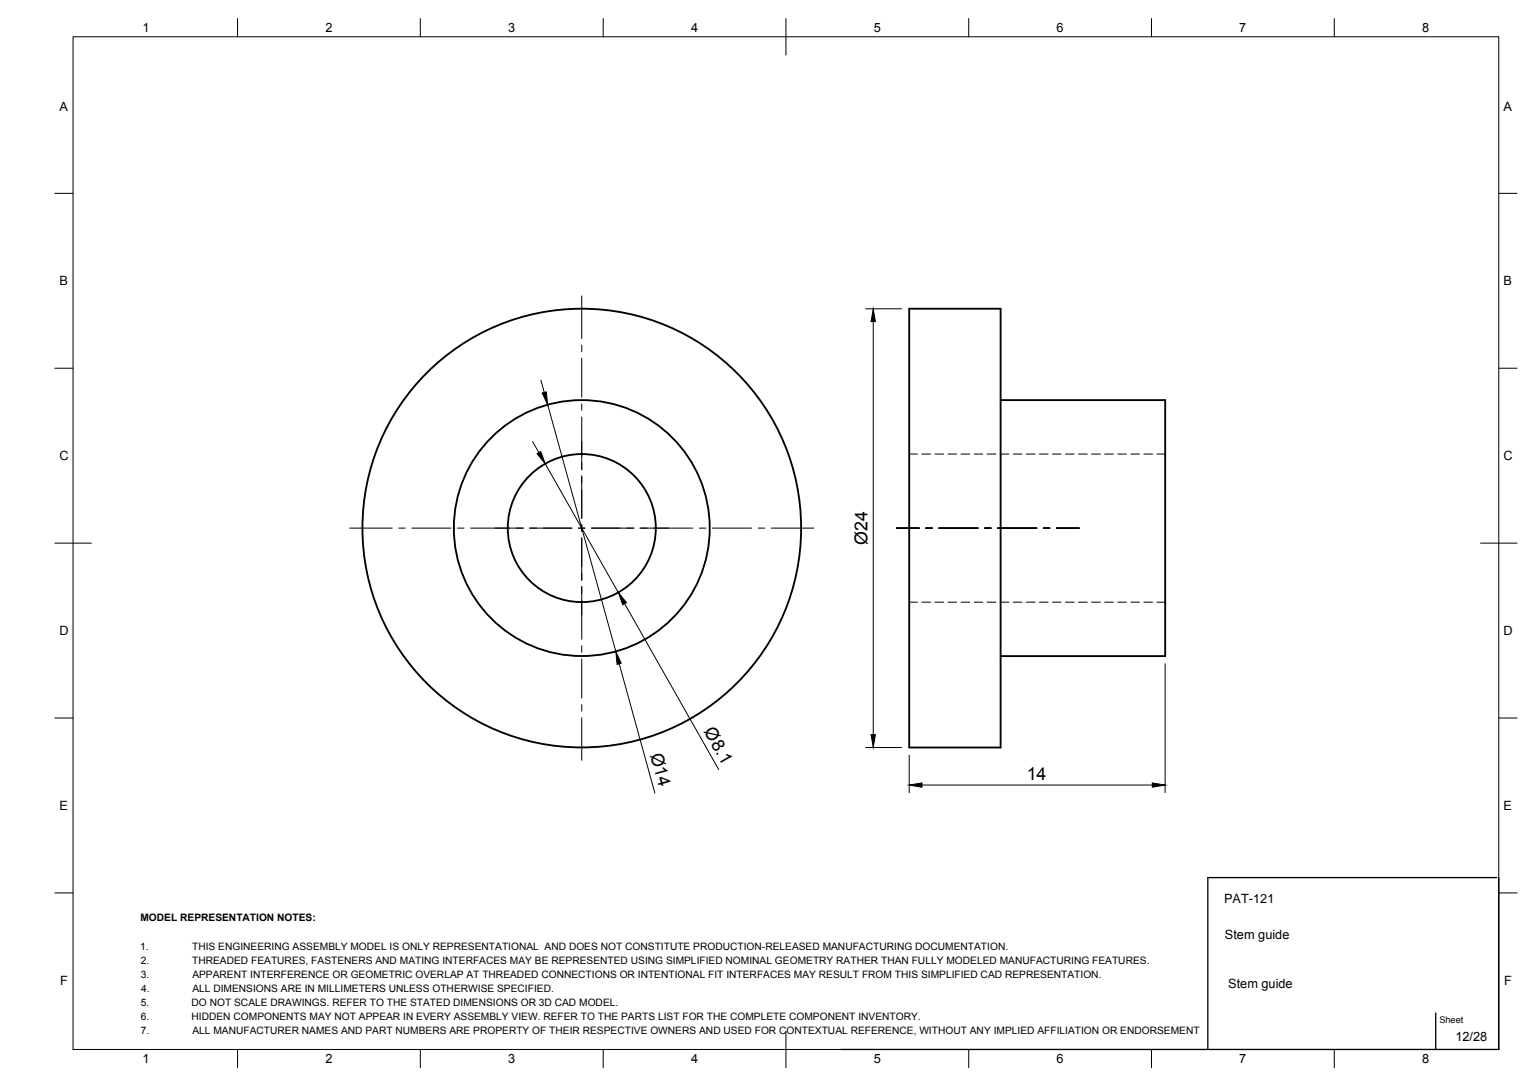
ISO-10303-21;
HEADER;
/* Generated by software containing ST-Developer
 * from STEP Tools, Inc. (www.steptools.com) 
 */

FILE_DESCRIPTION(
/* description */ ('Wall-mounted air drop station'),
/* implementation_level */ '2;1');

FILE_NAME(
/* name */ 'Stem guide.step',
/* time_stamp */ '2026-10-28T22:16:19-07:00',
/* author */ (''),
/* organization */ (''),
/* preprocessor_version */ 'ST-DEVELOPER v20.2',
/* originating_system */ 'Autodesk Translation Framework v15.17.0.0',
/* authorisation */ '');

FILE_SCHEMA (('AUTOMOTIVE_DESIGN { 1 0 10303 214 3 1 1 }'));
ENDSEC;

DATA;
#10=MECHANICAL_DESIGN_GEOMETRIC_PRESENTATION_REPRESENTATION('',(#352),#10517);
#294=SHAPE_REPRESENTATION_RELATIONSHIP('SRR','None',#10651,#323);
#323=ADVANCED_BREP_SHAPE_REPRESENTATION('',(#381),#10495);
#352=STYLED_ITEM('',(#10867),#381);
#381=MANIFOLD_SOLID_BREP('Body1',#5891);
#471=FACE_BOUND('',#1324,.T.);
#472=FACE_BOUND('',#1327,.T.);
#473=FACE_BOUND('',#1331,.T.);
#613=PLANE('',#6495);
#614=PLANE('',#6500);
#615=PLANE('',#6506);
#896=FACE_OUTER_BOUND('',#1323,.T.);
#897=FACE_OUTER_BOUND('',#1325,.T.);
#898=FACE_OUTER_BOUND('',#1326,.T.);
#899=FACE_OUTER_BOUND('',#1328,.T.);
#900=FACE_OUTER_BOUND('',#1329,.T.);
#901=FACE_OUTER_BOUND('',#1330,.T.);
#1323=EDGE_LOOP('',(#4591));
#1324=EDGE_LOOP('',(#4592));
#1325=EDGE_LOOP('',(#4593,#4594,#4595,#4596));
#1326=EDGE_LOOP('',(#4597));
#1327=EDGE_LOOP('',(#4598));
#1328=EDGE_LOOP('',(#4599,#4600,#4601,#4602));
#1329=EDGE_LOOP('',(#4603,#4604,#4605,#4606));
#1330=EDGE_LOOP('',(#4607));
#1331=EDGE_LOOP('',(#4608));
#1793=LINE('',#9441,#2257);
#1794=LINE('',#9447,#2258);
#1795=LINE('',#9451,#2259);
#2257=VECTOR('',#7655,1.2);
#2258=VECTOR('',#7662,0.405);
#2259=VECTOR('',#7667,0.7);
#2628=CIRCLE('',#6496,1.2);
#2629=CIRCLE('',#6497,0.7);
#2630=CIRCLE('',#6499,1.2);
#2631=CIRCLE('',#6501,0.405);
#2632=CIRCLE('',#6503,0.405);
#2633=CIRCLE('',#6505,0.7);
#2971=VERTEX_POINT('',#9434);
#2972=VERTEX_POINT('',#9436);
#2973=VERTEX_POINT('',#9439);
#2974=VERTEX_POINT('',#9443);
#2975=VERTEX_POINT('',#9446);
#2976=VERTEX_POINT('',#9450);
#3553=EDGE_CURVE('',#2971,#2971,#2628,.T.);
#3554=EDGE_CURVE('',#2972,#2972,#2629,.T.);
#3555=EDGE_CURVE('',#2973,#2973,#2630,.T.);
#3556=EDGE_CURVE('',#2973,#2971,#1793,.T.);
#3557=EDGE_CURVE('',#2974,#2974,#2631,.T.);
#3558=EDGE_CURVE('',#2974,#2975,#1794,.T.);
#3559=EDGE_CURVE('',#2975,#2975,#2632,.T.);
#3560=EDGE_CURVE('',#2972,#2976,#1795,.T.);
#3561=EDGE_CURVE('',#2976,#2976,#2633,.T.);
#4591=ORIENTED_EDGE('',*,*,#3553,.F.);
#4592=ORIENTED_EDGE('',*,*,#3554,.T.);
#4593=ORIENTED_EDGE('',*,*,#3555,.F.);
#4594=ORIENTED_EDGE('',*,*,#3556,.T.);
#4595=ORIENTED_EDGE('',*,*,#3553,.T.);
#4596=ORIENTED_EDGE('',*,*,#3556,.F.);
#4597=ORIENTED_EDGE('',*,*,#3555,.T.);
#4598=ORIENTED_EDGE('',*,*,#3557,.T.);
#4599=ORIENTED_EDGE('',*,*,#3557,.F.);
#4600=ORIENTED_EDGE('',*,*,#3558,.T.);
#4601=ORIENTED_EDGE('',*,*,#3559,.T.);
#4602=ORIENTED_EDGE('',*,*,#3558,.F.);
#4603=ORIENTED_EDGE('',*,*,#3554,.F.);
#4604=ORIENTED_EDGE('',*,*,#3560,.T.);
#4605=ORIENTED_EDGE('',*,*,#3561,.T.);
#4606=ORIENTED_EDGE('',*,*,#3560,.F.);
#4607=ORIENTED_EDGE('',*,*,#3561,.F.);
#4608=ORIENTED_EDGE('',*,*,#3559,.F.);
#5480=CYLINDRICAL_SURFACE('',#6498,1.2);
#5481=CYLINDRICAL_SURFACE('',#6502,0.405);
#5482=CYLINDRICAL_SURFACE('',#6504,0.7);
#5669=ADVANCED_FACE('',(#896,#471),#613,.F.);
#5670=ADVANCED_FACE('',(#897),#5480,.T.);
#5671=ADVANCED_FACE('',(#898,#472),#614,.T.);
#5672=ADVANCED_FACE('',(#899),#5481,.F.);
#5673=ADVANCED_FACE('',(#900),#5482,.T.);
#5674=ADVANCED_FACE('',(#901,#473),#615,.F.);
#5891=CLOSED_SHELL('',(#5669,#5670,#5671,#5672,#5673,#5674));
#6494=AXIS2_PLACEMENT_3D('',#9432,#7643,#7644);
#6495=AXIS2_PLACEMENT_3D('',#9433,#7645,#7646);
#6496=AXIS2_PLACEMENT_3D('',#9435,#7647,#7648);
#6497=AXIS2_PLACEMENT_3D('',#9437,#7649,#7650);
#6498=AXIS2_PLACEMENT_3D('',#9438,#7651,#7652);
#6499=AXIS2_PLACEMENT_3D('',#9440,#7653,#7654);
#6500=AXIS2_PLACEMENT_3D('',#9442,#7656,#7657);
#6501=AXIS2_PLACEMENT_3D('',#9444,#7658,#7659);
#6502=AXIS2_PLACEMENT_3D('',#9445,#7660,#7661);
#6503=AXIS2_PLACEMENT_3D('',#9448,#7663,#7664);
#6504=AXIS2_PLACEMENT_3D('',#9449,#7665,#7666);
#6505=AXIS2_PLACEMENT_3D('',#9452,#7668,#7669);
#6506=AXIS2_PLACEMENT_3D('',#9453,#7670,#7671);
#7643=DIRECTION('axis',(0.,0.,1.));
#7644=DIRECTION('refdir',(1.,0.,0.));
#7645=DIRECTION('center_axis',(0.,0.,1.));
#7646=DIRECTION('ref_axis',(1.,0.,0.));
#7647=DIRECTION('center_axis',(0.,0.,1.));
#7648=DIRECTION('ref_axis',(1.,0.,0.));
#7649=DIRECTION('center_axis',(0.,0.,1.));
#7650=DIRECTION('ref_axis',(1.,0.,0.));
#7651=DIRECTION('center_axis',(0.,0.,1.));
#7652=DIRECTION('ref_axis',(1.,0.,0.));
#7653=DIRECTION('center_axis',(0.,0.,1.));
#7654=DIRECTION('ref_axis',(1.,0.,0.));
#7655=DIRECTION('',(0.,0.,-1.));
#7656=DIRECTION('center_axis',(0.,0.,1.));
#7657=DIRECTION('ref_axis',(1.,0.,0.));
#7658=DIRECTION('center_axis',(0.,0.,-1.));
#7659=DIRECTION('ref_axis',(1.,0.,0.));
#7660=DIRECTION('center_axis',(0.,0.,1.));
#7661=DIRECTION('ref_axis',(1.,0.,0.));
#7662=DIRECTION('',(0.,0.,-1.));
#7663=DIRECTION('center_axis',(0.,0.,-1.));
#7664=DIRECTION('ref_axis',(1.,0.,0.));
#7665=DIRECTION('center_axis',(0.,0.,1.));
#7666=DIRECTION('ref_axis',(1.,0.,0.));
#7667=DIRECTION('',(0.,0.,-1.));
#7668=DIRECTION('center_axis',(0.,0.,1.));
#7669=DIRECTION('ref_axis',(1.,0.,0.));
#7670=DIRECTION('center_axis',(0.,0.,1.));
#7671=DIRECTION('ref_axis',(1.,0.,0.));
#9432=CARTESIAN_POINT('',(0.,0.,0.));
#9433=CARTESIAN_POINT('Origin',(0.,0.,7.5));
#9434=CARTESIAN_POINT('',(-1.2,-1.46957615897682E-16,7.5));
#9435=CARTESIAN_POINT('Origin',(0.,0.,7.5));
#9436=CARTESIAN_POINT('',(-0.7,-8.57252759403147E-17,7.5));
#9437=CARTESIAN_POINT('Origin',(0.,0.,7.5));
#9438=CARTESIAN_POINT('Origin',(0.,0.,7.5));
#9439=CARTESIAN_POINT('',(-1.2,-1.46957615897682E-16,8.));
#9440=CARTESIAN_POINT('Origin',(0.,0.,8.));
#9441=CARTESIAN_POINT('',(-1.2,-1.46957615897682E-16,7.5));
#9442=CARTESIAN_POINT('Origin',(0.,0.,8.));
#9443=CARTESIAN_POINT('',(-0.405,-4.95981953654678E-17,8.));
#9444=CARTESIAN_POINT('Origin',(0.,0.,8.));
#9445=CARTESIAN_POINT('Origin',(0.,0.,6.6));
#9446=CARTESIAN_POINT('',(-0.405,-4.95981953654678E-17,6.6));
#9447=CARTESIAN_POINT('',(-0.405,-4.95981953654678E-17,6.6));
#9448=CARTESIAN_POINT('Origin',(0.,0.,6.6));
#9449=CARTESIAN_POINT('Origin',(0.,0.,6.6));
#9450=CARTESIAN_POINT('',(-0.7,-8.57252759403147E-17,6.6));
#9451=CARTESIAN_POINT('',(-0.7,-8.57252759403147E-17,6.6));
#9452=CARTESIAN_POINT('Origin',(0.,0.,6.6));
#9453=CARTESIAN_POINT('Origin',(0.,0.,6.6));
#10462=UNCERTAINTY_MEASURE_WITH_UNIT(LENGTH_MEASURE(0.001),#10518,
'DISTANCE_ACCURACY_VALUE',
'Maximum model space distance between geometric entities at asserted c
onnectivities');
#10484=UNCERTAINTY_MEASURE_WITH_UNIT(LENGTH_MEASURE(0.001),#10518,
'DISTANCE_ACCURACY_VALUE',
'Maximum model space distance between geometric entities at asserted c
onnectivities');
#10495=(
GEOMETRIC_REPRESENTATION_CONTEXT(3)
GLOBAL_UNCERTAINTY_ASSIGNED_CONTEXT((#10462))
GLOBAL_UNIT_ASSIGNED_CONTEXT((#10518,#10520,#10521))
REPRESENTATION_CONTEXT('','3D')
);
#10517=(
GEOMETRIC_REPRESENTATION_CONTEXT(3)
GLOBAL_UNCERTAINTY_ASSIGNED_CONTEXT((#10484))
GLOBAL_UNIT_ASSIGNED_CONTEXT((#10518,#10520,#10521))
REPRESENTATION_CONTEXT('','3D')
);
#10518=(
LENGTH_UNIT()
NAMED_UNIT(*)
SI_UNIT(.CENTI.,.METRE.)
);
#10520=(
NAMED_UNIT(*)
PLANE_ANGLE_UNIT()
SI_UNIT($,.RADIAN.)
);
#10521=(
NAMED_UNIT(*)
SI_UNIT($,.STERADIAN.)
SOLID_ANGLE_UNIT()
);
#10532=SHAPE_DEFINITION_REPRESENTATION(#10564,#10651);
#10564=PRODUCT_DEFINITION_SHAPE('',$,#10684);
#10651=SHAPE_REPRESENTATION('',(#6494),#10495);
#10673=PRODUCT_DEFINITION_CONTEXT('part definition',#10771,'design');
#10684=PRODUCT_DEFINITION('Stem guide','Stem guide',#10716,#10673);
#10716=PRODUCT_DEFINITION_FORMATION('',$,#10783);
#10771=APPLICATION_CONTEXT(
'Core Data for Automotive Mechanical Design Process');
#10772=PRODUCT_CONTEXT('part definition',#10771,'mechanical');
#10783=PRODUCT('Stem guide','Stem guide','Stem guide',(#10772));
#10861=COLOUR_RGB('Sky Blue',0.24,0.69,0.87);
#10862=FILL_AREA_STYLE_COLOUR('',#10861);
#10863=FILL_AREA_STYLE('',(#10862));
#10864=SURFACE_STYLE_FILL_AREA(#10863);
#10865=SURFACE_SIDE_STYLE('',(#10864));
#10866=SURFACE_STYLE_USAGE(.BOTH.,#10865);
#10867=PRESENTATION_STYLE_ASSIGNMENT((#10866));
ENDSEC;
END-ISO-10303-21;
